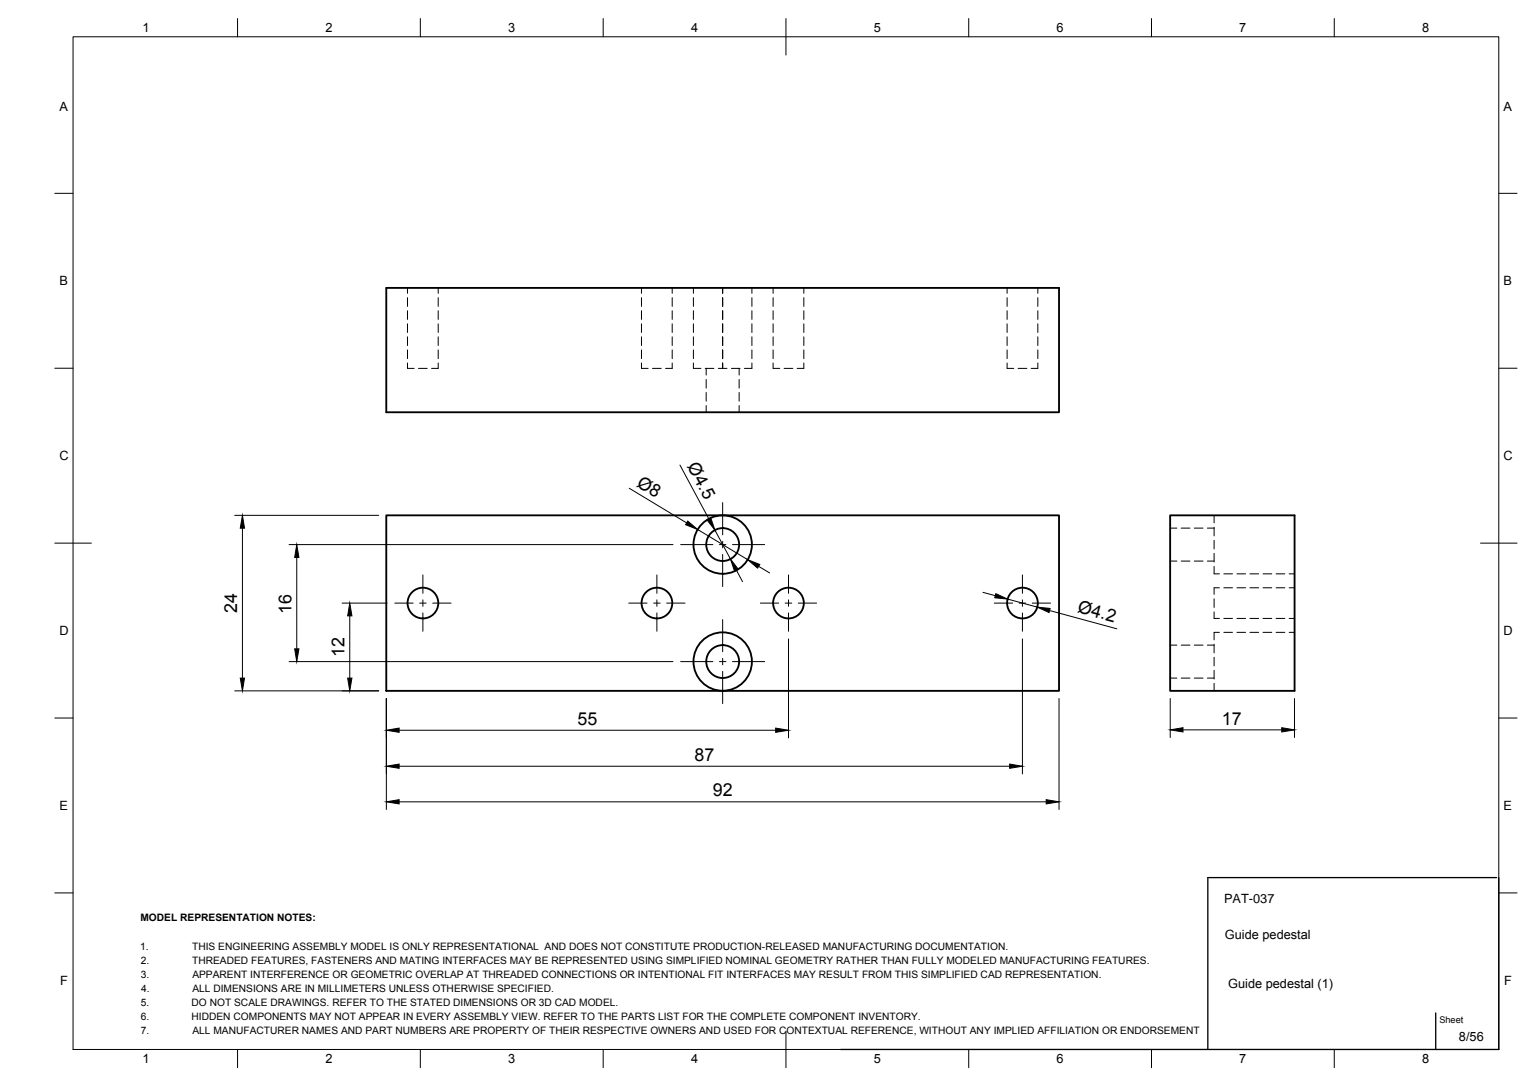
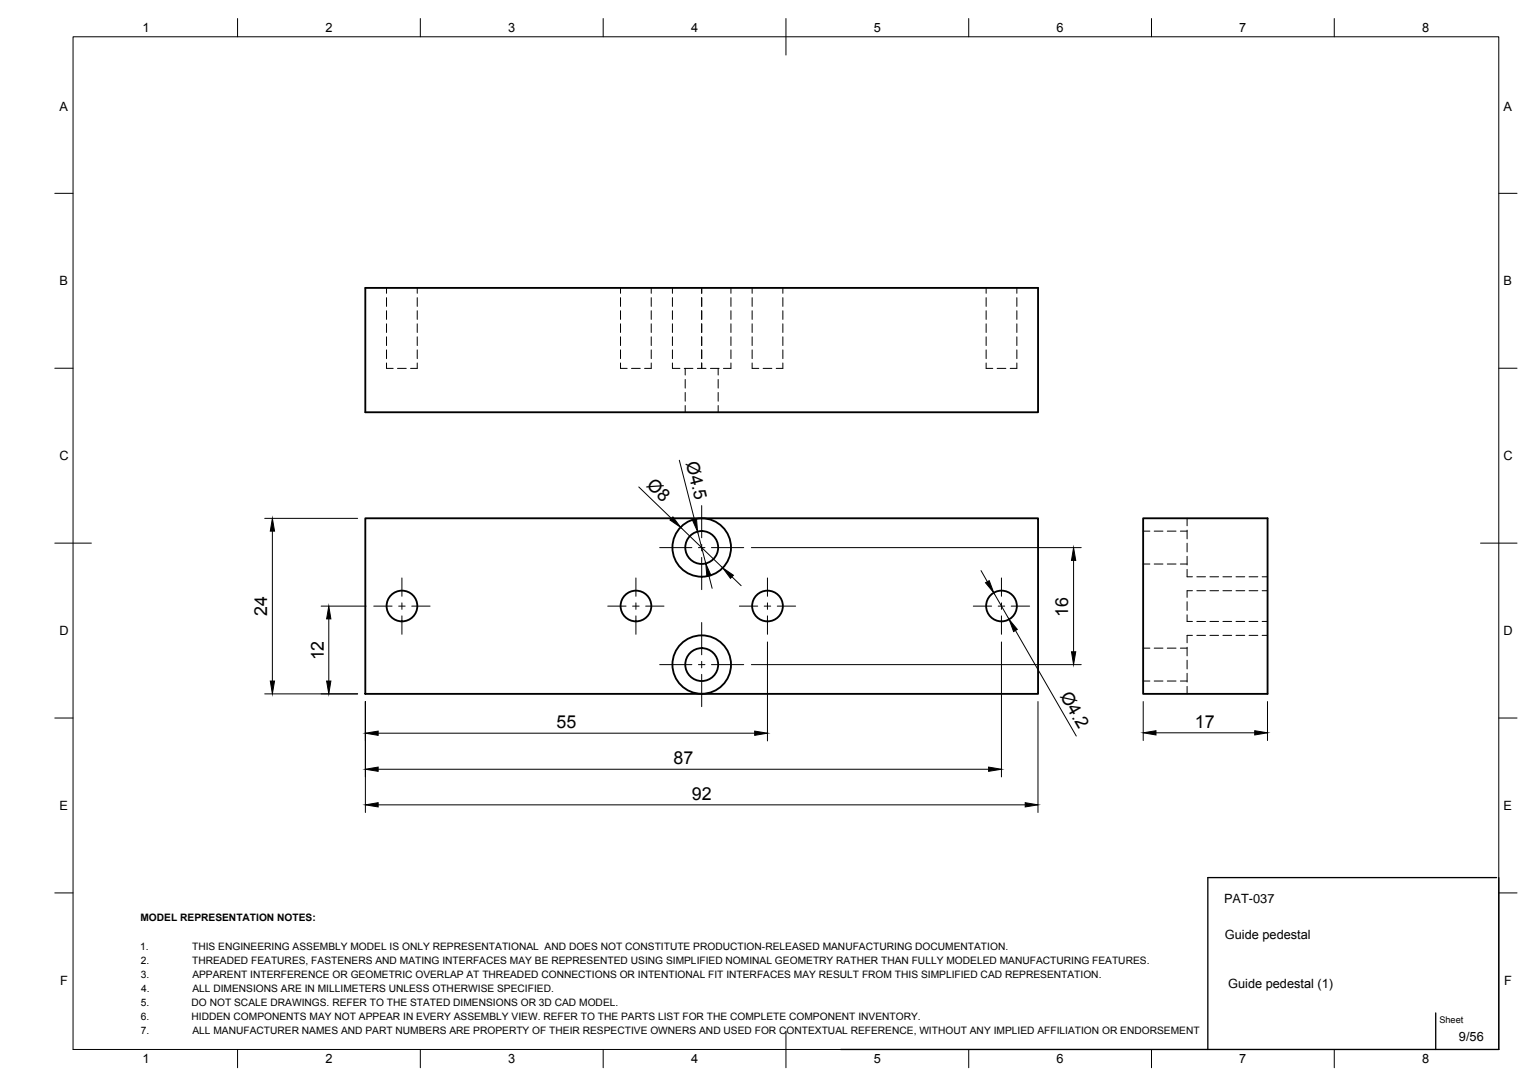
ISO-10303-21;
HEADER;
/* Generated by software containing ST-Developer
 * from STEP Tools, Inc. (www.steptools.com) 
 */

FILE_DESCRIPTION(
/* description */ ('Flywheel Crank-Slider'),
/* implementation_level */ '2;1');

FILE_NAME(
/* name */ 'Guide pedestal.step',
/* time_stamp */ '2026-10-28T03:23:13-07:00',
/* author */ (''),
/* organization */ (''),
/* preprocessor_version */ 'ST-DEVELOPER v20.2',
/* originating_system */ 'Autodesk Translation Framework v15.17.0.0',
/* authorisation */ '');

FILE_SCHEMA (('AUTOMOTIVE_DESIGN { 1 0 10303 214 3 1 1 }'));
ENDSEC;

DATA;
#10=MECHANICAL_DESIGN_GEOMETRIC_PRESENTATION_REPRESENTATION('',(#675),#17322);
#571=SHAPE_REPRESENTATION_RELATIONSHIP('SRR','None',#17567,#623);
#623=ADVANCED_BREP_SHAPE_REPRESENTATION('',(#736),#17271);
#675=STYLED_ITEM('',(#17945),#736);
#736=MANIFOLD_SOLID_BREP('Body1',#9053);
#845=FACE_BOUND('',#1996,.T.);
#846=FACE_BOUND('',#1999,.T.);
#847=FACE_BOUND('',#2001,.T.);
#848=FACE_BOUND('',#2002,.T.);
#849=FACE_BOUND('',#2003,.T.);
#850=FACE_BOUND('',#2004,.T.);
#851=FACE_BOUND('',#2020,.T.);
#852=FACE_BOUND('',#2021,.T.);
#1049=PLANE('',#9859);
#1050=PLANE('',#9864);
#1051=PLANE('',#9866);
#1052=PLANE('',#9877);
#1053=PLANE('',#9880);
#1054=PLANE('',#9883);
#1055=PLANE('',#9886);
#1056=PLANE('',#9887);
#1057=PLANE('',#9888);
#1058=PLANE('',#9889);
#1059=PLANE('',#9890);
#1060=PLANE('',#9891);
#1398=FACE_OUTER_BOUND('',#1993,.T.);
#1399=FACE_OUTER_BOUND('',#1994,.T.);
#1400=FACE_OUTER_BOUND('',#1995,.T.);
#1401=FACE_OUTER_BOUND('',#1997,.T.);
#1402=FACE_OUTER_BOUND('',#1998,.T.);
#1403=FACE_OUTER_BOUND('',#2000,.T.);
#1404=FACE_OUTER_BOUND('',#2005,.T.);
#1405=FACE_OUTER_BOUND('',#2006,.T.);
#1406=FACE_OUTER_BOUND('',#2007,.T.);
#1407=FACE_OUTER_BOUND('',#2008,.T.);
#1408=FACE_OUTER_BOUND('',#2009,.T.);
#1409=FACE_OUTER_BOUND('',#2010,.T.);
#1410=FACE_OUTER_BOUND('',#2011,.T.);
#1411=FACE_OUTER_BOUND('',#2012,.T.);
#1412=FACE_OUTER_BOUND('',#2013,.T.);
#1413=FACE_OUTER_BOUND('',#2014,.T.);
#1414=FACE_OUTER_BOUND('',#2015,.T.);
#1415=FACE_OUTER_BOUND('',#2016,.T.);
#1416=FACE_OUTER_BOUND('',#2017,.T.);
#1417=FACE_OUTER_BOUND('',#2018,.T.);
#1418=FACE_OUTER_BOUND('',#2019,.T.);
#1993=EDGE_LOOP('',(#6434,#6435,#6436,#6437));
#1994=EDGE_LOOP('',(#6438,#6439,#6440,#6441));
#1995=EDGE_LOOP('',(#6442));
#1996=EDGE_LOOP('',(#6443));
#1997=EDGE_LOOP('',(#6444,#6445,#6446,#6447));
#1998=EDGE_LOOP('',(#6448,#6449));
#1999=EDGE_LOOP('',(#6450));
#2000=EDGE_LOOP('',(#6451,#6452,#6453,#6454,#6455,#6456,#6457,#6458,#6459));
#2001=EDGE_LOOP('',(#6460));
#2002=EDGE_LOOP('',(#6461));
#2003=EDGE_LOOP('',(#6462));
#2004=EDGE_LOOP('',(#6463));
#2005=EDGE_LOOP('',(#6464,#6465,#6466,#6467));
#2006=EDGE_LOOP('',(#6468,#6469,#6470,#6471));
#2007=EDGE_LOOP('',(#6472,#6473,#6474,#6475));
#2008=EDGE_LOOP('',(#6476));
#2009=EDGE_LOOP('',(#6477,#6478,#6479,#6480));
#2010=EDGE_LOOP('',(#6481));
#2011=EDGE_LOOP('',(#6482,#6483,#6484,#6485));
#2012=EDGE_LOOP('',(#6486));
#2013=EDGE_LOOP('',(#6487,#6488,#6489,#6490));
#2014=EDGE_LOOP('',(#6491));
#2015=EDGE_LOOP('',(#6492,#6493,#6494,#6495));
#2016=EDGE_LOOP('',(#6496,#6497,#6498,#6499,#6500,#6501,#6502));
#2017=EDGE_LOOP('',(#6503,#6504,#6505,#6506));
#2018=EDGE_LOOP('',(#6507,#6508,#6509,#6510,#6511,#6512,#6513));
#2019=EDGE_LOOP('',(#6514,#6515,#6516,#6517));
#2020=EDGE_LOOP('',(#6518));
#2021=EDGE_LOOP('',(#6519));
#2692=LINE('',#14082,#3303);
#2693=LINE('',#14086,#3304);
#2694=LINE('',#14092,#3305);
#2695=LINE('',#14094,#3306);
#2696=LINE('',#14100,#3307);
#2697=LINE('',#14107,#3308);
#2698=LINE('',#14109,#3309);
#2699=LINE('',#14111,#3310);
#2700=LINE('',#14112,#3311);
#2701=LINE('',#14114,#3312);
#2702=LINE('',#14115,#3313);
#2703=LINE('',#14127,#3314);
#2704=LINE('',#14131,#3315);
#2705=LINE('',#14135,#3316);
#2706=LINE('',#14140,#3317);
#2707=LINE('',#14145,#3318);
#2708=LINE('',#14150,#3319);
#2709=LINE('',#14155,#3320);
#2710=LINE('',#14156,#3321);
#2711=LINE('',#14157,#3322);
#2712=LINE('',#14160,#3323);
#2713=LINE('',#14161,#3324);
#2714=LINE('',#14164,#3325);
#2715=LINE('',#14165,#3326);
#2716=LINE('',#14167,#3327);
#3303=VECTOR('',#11244,0.4);
#3304=VECTOR('',#11247,1.);
#3305=VECTOR('',#11254,1.);
#3306=VECTOR('',#11257,1.);
#3307=VECTOR('',#11266,1.);
#3308=VECTOR('',#11275,1.);
#3309=VECTOR('',#11276,1.);
#3310=VECTOR('',#11277,1.);
#3311=VECTOR('',#11278,1.);
#3312=VECTOR('',#11279,1.);
#3313=VECTOR('',#11280,1.);
#3314=VECTOR('',#11293,0.225);
#3315=VECTOR('',#11298,0.225);
#3316=VECTOR('',#11303,0.21);
#3317=VECTOR('',#11310,0.21);
#3318=VECTOR('',#11317,0.21);
#3319=VECTOR('',#11324,0.21);
#3320=VECTOR('',#11329,1.);
#3321=VECTOR('',#11330,1.);
#3322=VECTOR('',#11331,1.);
#3323=VECTOR('',#11334,1.);
#3324=VECTOR('',#11335,1.);
#3325=VECTOR('',#11338,1.);
#3326=VECTOR('',#11339,1.);
#3327=VECTOR('',#11342,1.);
#3918=CIRCLE('',#9854,0.4);
#3919=CIRCLE('',#9855,0.4);
#3920=CIRCLE('',#9857,0.4);
#3921=CIRCLE('',#9858,0.4);
#3922=CIRCLE('',#9860,0.225);
#3923=CIRCLE('',#9862,0.4);
#3924=CIRCLE('',#9863,0.4);
#3925=CIRCLE('',#9865,0.225);
#3926=CIRCLE('',#9867,0.21);
#3927=CIRCLE('',#9868,0.21);
#3928=CIRCLE('',#9869,0.21);
#3929=CIRCLE('',#9870,0.21);
#3930=CIRCLE('',#9872,0.225);
#3931=CIRCLE('',#9874,0.225);
#3932=CIRCLE('',#9876,0.21);
#3933=CIRCLE('',#9879,0.21);
#3934=CIRCLE('',#9882,0.21);
#3935=CIRCLE('',#9885,0.21);
#4381=VERTEX_POINT('',#14080);
#4382=VERTEX_POINT('',#14081);
#4383=VERTEX_POINT('',#14083);
#4384=VERTEX_POINT('',#14085);
#4385=VERTEX_POINT('',#14089);
#4386=VERTEX_POINT('',#14091);
#4387=VERTEX_POINT('',#14096);
#4388=VERTEX_POINT('',#14103);
#4389=VERTEX_POINT('',#14106);
#4390=VERTEX_POINT('',#14108);
#4391=VERTEX_POINT('',#14110);
#4392=VERTEX_POINT('',#14113);
#4393=VERTEX_POINT('',#14116);
#4394=VERTEX_POINT('',#14118);
#4395=VERTEX_POINT('',#14120);
#4396=VERTEX_POINT('',#14122);
#4397=VERTEX_POINT('',#14125);
#4398=VERTEX_POINT('',#14129);
#4399=VERTEX_POINT('',#14133);
#4400=VERTEX_POINT('',#14138);
#4401=VERTEX_POINT('',#14143);
#4402=VERTEX_POINT('',#14148);
#4403=VERTEX_POINT('',#14153);
#4404=VERTEX_POINT('',#14154);
#4405=VERTEX_POINT('',#14159);
#4406=VERTEX_POINT('',#14163);
#5174=EDGE_CURVE('',#4381,#4382,#2692,.T.);
#5175=EDGE_CURVE('',#4383,#4381,#3918,.T.);
#5176=EDGE_CURVE('',#4383,#4384,#2693,.T.);
#5177=EDGE_CURVE('',#4382,#4384,#3919,.T.);
#5178=EDGE_CURVE('',#4385,#4385,#3920,.T.);
#5179=EDGE_CURVE('',#4385,#4386,#2694,.T.);
#5180=EDGE_CURVE('',#4386,#4386,#3921,.T.);
#5181=EDGE_CURVE('',#4385,#4386,#2695,.T.);
#5182=EDGE_CURVE('',#4387,#4387,#3922,.T.);
#5183=EDGE_CURVE('',#4384,#4382,#3923,.T.);
#5184=EDGE_CURVE('',#4383,#4384,#2696,.T.);
#5185=EDGE_CURVE('',#4381,#4383,#3924,.T.);
#5186=EDGE_CURVE('',#4388,#4388,#3925,.T.);
#5187=EDGE_CURVE('',#4389,#4386,#2697,.T.);
#5188=EDGE_CURVE('',#4386,#4390,#2698,.T.);
#5189=EDGE_CURVE('',#4390,#4391,#2699,.T.);
#5190=EDGE_CURVE('',#4391,#4384,#2700,.T.);
#5191=EDGE_CURVE('',#4384,#4392,#2701,.T.);
#5192=EDGE_CURVE('',#4392,#4389,#2702,.T.);
#5193=EDGE_CURVE('',#4393,#4393,#3926,.T.);
#5194=EDGE_CURVE('',#4394,#4394,#3927,.T.);
#5195=EDGE_CURVE('',#4395,#4395,#3928,.T.);
#5196=EDGE_CURVE('',#4396,#4396,#3929,.T.);
#5197=EDGE_CURVE('',#4397,#4397,#3930,.T.);
#5198=EDGE_CURVE('',#4397,#4387,#2703,.T.);
#5199=EDGE_CURVE('',#4398,#4398,#3931,.T.);
#5200=EDGE_CURVE('',#4398,#4388,#2704,.T.);
#5201=EDGE_CURVE('',#4399,#4399,#3932,.T.);
#5202=EDGE_CURVE('',#4399,#4396,#2705,.T.);
#5203=EDGE_CURVE('',#4400,#4400,#3933,.T.);
#5204=EDGE_CURVE('',#4400,#4395,#2706,.T.);
#5205=EDGE_CURVE('',#4401,#4401,#3934,.T.);
#5206=EDGE_CURVE('',#4401,#4394,#2707,.T.);
#5207=EDGE_CURVE('',#4402,#4402,#3935,.T.);
#5208=EDGE_CURVE('',#4402,#4393,#2708,.T.);
#5209=EDGE_CURVE('',#4403,#4404,#2709,.T.);
#5210=EDGE_CURVE('',#4404,#4389,#2710,.T.);
#5211=EDGE_CURVE('',#4403,#4392,#2711,.T.);
#5212=EDGE_CURVE('',#4405,#4403,#2712,.T.);
#5213=EDGE_CURVE('',#4405,#4391,#2713,.T.);
#5214=EDGE_CURVE('',#4406,#4405,#2714,.T.);
#5215=EDGE_CURVE('',#4406,#4390,#2715,.T.);
#5216=EDGE_CURVE('',#4404,#4406,#2716,.T.);
#6434=ORIENTED_EDGE('',*,*,#5174,.F.);
#6435=ORIENTED_EDGE('',*,*,#5175,.F.);
#6436=ORIENTED_EDGE('',*,*,#5176,.T.);
#6437=ORIENTED_EDGE('',*,*,#5177,.F.);
#6438=ORIENTED_EDGE('',*,*,#5178,.F.);
#6439=ORIENTED_EDGE('',*,*,#5179,.T.);
#6440=ORIENTED_EDGE('',*,*,#5180,.F.);
#6441=ORIENTED_EDGE('',*,*,#5181,.F.);
#6442=ORIENTED_EDGE('',*,*,#5178,.T.);
#6443=ORIENTED_EDGE('',*,*,#5182,.F.);
#6444=ORIENTED_EDGE('',*,*,#5174,.T.);
#6445=ORIENTED_EDGE('',*,*,#5183,.F.);
#6446=ORIENTED_EDGE('',*,*,#5184,.F.);
#6447=ORIENTED_EDGE('',*,*,#5185,.F.);
#6448=ORIENTED_EDGE('',*,*,#5175,.T.);
#6449=ORIENTED_EDGE('',*,*,#5185,.T.);
#6450=ORIENTED_EDGE('',*,*,#5186,.F.);
#6451=ORIENTED_EDGE('',*,*,#5187,.T.);
#6452=ORIENTED_EDGE('',*,*,#5180,.T.);
#6453=ORIENTED_EDGE('',*,*,#5188,.T.);
#6454=ORIENTED_EDGE('',*,*,#5189,.T.);
#6455=ORIENTED_EDGE('',*,*,#5190,.T.);
#6456=ORIENTED_EDGE('',*,*,#5183,.T.);
#6457=ORIENTED_EDGE('',*,*,#5177,.T.);
#6458=ORIENTED_EDGE('',*,*,#5191,.T.);
#6459=ORIENTED_EDGE('',*,*,#5192,.T.);
#6460=ORIENTED_EDGE('',*,*,#5193,.T.);
#6461=ORIENTED_EDGE('',*,*,#5194,.T.);
#6462=ORIENTED_EDGE('',*,*,#5195,.T.);
#6463=ORIENTED_EDGE('',*,*,#5196,.T.);
#6464=ORIENTED_EDGE('',*,*,#5197,.F.);
#6465=ORIENTED_EDGE('',*,*,#5198,.T.);
#6466=ORIENTED_EDGE('',*,*,#5182,.T.);
#6467=ORIENTED_EDGE('',*,*,#5198,.F.);
#6468=ORIENTED_EDGE('',*,*,#5199,.F.);
#6469=ORIENTED_EDGE('',*,*,#5200,.T.);
#6470=ORIENTED_EDGE('',*,*,#5186,.T.);
#6471=ORIENTED_EDGE('',*,*,#5200,.F.);
#6472=ORIENTED_EDGE('',*,*,#5201,.F.);
#6473=ORIENTED_EDGE('',*,*,#5202,.T.);
#6474=ORIENTED_EDGE('',*,*,#5196,.F.);
#6475=ORIENTED_EDGE('',*,*,#5202,.F.);
#6476=ORIENTED_EDGE('',*,*,#5201,.T.);
#6477=ORIENTED_EDGE('',*,*,#5203,.F.);
#6478=ORIENTED_EDGE('',*,*,#5204,.T.);
#6479=ORIENTED_EDGE('',*,*,#5195,.F.);
#6480=ORIENTED_EDGE('',*,*,#5204,.F.);
#6481=ORIENTED_EDGE('',*,*,#5203,.T.);
#6482=ORIENTED_EDGE('',*,*,#5205,.F.);
#6483=ORIENTED_EDGE('',*,*,#5206,.T.);
#6484=ORIENTED_EDGE('',*,*,#5194,.F.);
#6485=ORIENTED_EDGE('',*,*,#5206,.F.);
#6486=ORIENTED_EDGE('',*,*,#5205,.T.);
#6487=ORIENTED_EDGE('',*,*,#5207,.F.);
#6488=ORIENTED_EDGE('',*,*,#5208,.T.);
#6489=ORIENTED_EDGE('',*,*,#5193,.F.);
#6490=ORIENTED_EDGE('',*,*,#5208,.F.);
#6491=ORIENTED_EDGE('',*,*,#5207,.T.);
#6492=ORIENTED_EDGE('',*,*,#5209,.T.);
#6493=ORIENTED_EDGE('',*,*,#5210,.T.);
#6494=ORIENTED_EDGE('',*,*,#5192,.F.);
#6495=ORIENTED_EDGE('',*,*,#5211,.F.);
#6496=ORIENTED_EDGE('',*,*,#5212,.T.);
#6497=ORIENTED_EDGE('',*,*,#5211,.T.);
#6498=ORIENTED_EDGE('',*,*,#5191,.F.);
#6499=ORIENTED_EDGE('',*,*,#5176,.F.);
#6500=ORIENTED_EDGE('',*,*,#5184,.T.);
#6501=ORIENTED_EDGE('',*,*,#5190,.F.);
#6502=ORIENTED_EDGE('',*,*,#5213,.F.);
#6503=ORIENTED_EDGE('',*,*,#5214,.T.);
#6504=ORIENTED_EDGE('',*,*,#5213,.T.);
#6505=ORIENTED_EDGE('',*,*,#5189,.F.);
#6506=ORIENTED_EDGE('',*,*,#5215,.F.);
#6507=ORIENTED_EDGE('',*,*,#5216,.T.);
#6508=ORIENTED_EDGE('',*,*,#5215,.T.);
#6509=ORIENTED_EDGE('',*,*,#5188,.F.);
#6510=ORIENTED_EDGE('',*,*,#5179,.F.);
#6511=ORIENTED_EDGE('',*,*,#5181,.T.);
#6512=ORIENTED_EDGE('',*,*,#5187,.F.);
#6513=ORIENTED_EDGE('',*,*,#5210,.F.);
#6514=ORIENTED_EDGE('',*,*,#5216,.F.);
#6515=ORIENTED_EDGE('',*,*,#5209,.F.);
#6516=ORIENTED_EDGE('',*,*,#5212,.F.);
#6517=ORIENTED_EDGE('',*,*,#5214,.F.);
#6518=ORIENTED_EDGE('',*,*,#5197,.T.);
#6519=ORIENTED_EDGE('',*,*,#5199,.T.);
#8370=CYLINDRICAL_SURFACE('',#9853,0.4);
#8371=CYLINDRICAL_SURFACE('',#9856,0.4);
#8372=CYLINDRICAL_SURFACE('',#9861,0.4);
#8373=CYLINDRICAL_SURFACE('',#9871,0.225);
#8374=CYLINDRICAL_SURFACE('',#9873,0.225);
#8375=CYLINDRICAL_SURFACE('',#9875,0.21);
#8376=CYLINDRICAL_SURFACE('',#9878,0.21);
#8377=CYLINDRICAL_SURFACE('',#9881,0.21);
#8378=CYLINDRICAL_SURFACE('',#9884,0.21);
#8589=ADVANCED_FACE('',(#1398),#8370,.F.);
#8590=ADVANCED_FACE('',(#1399),#8371,.F.);
#8591=ADVANCED_FACE('',(#1400,#845),#1049,.T.);
#8592=ADVANCED_FACE('',(#1401),#8372,.F.);
#8593=ADVANCED_FACE('',(#1402,#846),#1050,.T.);
#8594=ADVANCED_FACE('',(#1403,#847,#848,#849,#850),#1051,.T.);
#8595=ADVANCED_FACE('',(#1404),#8373,.F.);
#8596=ADVANCED_FACE('',(#1405),#8374,.F.);
#8597=ADVANCED_FACE('',(#1406),#8375,.F.);
#8598=ADVANCED_FACE('',(#1407),#1052,.T.);
#8599=ADVANCED_FACE('',(#1408),#8376,.F.);
#8600=ADVANCED_FACE('',(#1409),#1053,.T.);
#8601=ADVANCED_FACE('',(#1410),#8377,.F.);
#8602=ADVANCED_FACE('',(#1411),#1054,.T.);
#8603=ADVANCED_FACE('',(#1412),#8378,.F.);
#8604=ADVANCED_FACE('',(#1413),#1055,.T.);
#8605=ADVANCED_FACE('',(#1414),#1056,.T.);
#8606=ADVANCED_FACE('',(#1415),#1057,.T.);
#8607=ADVANCED_FACE('',(#1416),#1058,.T.);
#8608=ADVANCED_FACE('',(#1417),#1059,.T.);
#8609=ADVANCED_FACE('',(#1418,#851,#852),#1060,.F.);
#9053=CLOSED_SHELL('',(#8589,#8590,#8591,#8592,#8593,#8594,#8595,#8596,
#8597,#8598,#8599,#8600,#8601,#8602,#8603,#8604,#8605,#8606,#8607,#8608,
#8609));
#9852=AXIS2_PLACEMENT_3D('',#14078,#11240,#11241);
#9853=AXIS2_PLACEMENT_3D('',#14079,#11242,#11243);
#9854=AXIS2_PLACEMENT_3D('',#14084,#11245,#11246);
#9855=AXIS2_PLACEMENT_3D('',#14087,#11248,#11249);
#9856=AXIS2_PLACEMENT_3D('',#14088,#11250,#11251);
#9857=AXIS2_PLACEMENT_3D('',#14090,#11252,#11253);
#9858=AXIS2_PLACEMENT_3D('',#14093,#11255,#11256);
#9859=AXIS2_PLACEMENT_3D('',#14095,#11258,#11259);
#9860=AXIS2_PLACEMENT_3D('',#14097,#11260,#11261);
#9861=AXIS2_PLACEMENT_3D('',#14098,#11262,#11263);
#9862=AXIS2_PLACEMENT_3D('',#14099,#11264,#11265);
#9863=AXIS2_PLACEMENT_3D('',#14101,#11267,#11268);
#9864=AXIS2_PLACEMENT_3D('',#14102,#11269,#11270);
#9865=AXIS2_PLACEMENT_3D('',#14104,#11271,#11272);
#9866=AXIS2_PLACEMENT_3D('',#14105,#11273,#11274);
#9867=AXIS2_PLACEMENT_3D('',#14117,#11281,#11282);
#9868=AXIS2_PLACEMENT_3D('',#14119,#11283,#11284);
#9869=AXIS2_PLACEMENT_3D('',#14121,#11285,#11286);
#9870=AXIS2_PLACEMENT_3D('',#14123,#11287,#11288);
#9871=AXIS2_PLACEMENT_3D('',#14124,#11289,#11290);
#9872=AXIS2_PLACEMENT_3D('',#14126,#11291,#11292);
#9873=AXIS2_PLACEMENT_3D('',#14128,#11294,#11295);
#9874=AXIS2_PLACEMENT_3D('',#14130,#11296,#11297);
#9875=AXIS2_PLACEMENT_3D('',#14132,#11299,#11300);
#9876=AXIS2_PLACEMENT_3D('',#14134,#11301,#11302);
#9877=AXIS2_PLACEMENT_3D('',#14136,#11304,#11305);
#9878=AXIS2_PLACEMENT_3D('',#14137,#11306,#11307);
#9879=AXIS2_PLACEMENT_3D('',#14139,#11308,#11309);
#9880=AXIS2_PLACEMENT_3D('',#14141,#11311,#11312);
#9881=AXIS2_PLACEMENT_3D('',#14142,#11313,#11314);
#9882=AXIS2_PLACEMENT_3D('',#14144,#11315,#11316);
#9883=AXIS2_PLACEMENT_3D('',#14146,#11318,#11319);
#9884=AXIS2_PLACEMENT_3D('',#14147,#11320,#11321);
#9885=AXIS2_PLACEMENT_3D('',#14149,#11322,#11323);
#9886=AXIS2_PLACEMENT_3D('',#14151,#11325,#11326);
#9887=AXIS2_PLACEMENT_3D('',#14152,#11327,#11328);
#9888=AXIS2_PLACEMENT_3D('',#14158,#11332,#11333);
#9889=AXIS2_PLACEMENT_3D('',#14162,#11336,#11337);
#9890=AXIS2_PLACEMENT_3D('',#14166,#11340,#11341);
#9891=AXIS2_PLACEMENT_3D('',#14168,#11343,#11344);
#11240=DIRECTION('axis',(0.,0.,1.));
#11241=DIRECTION('refdir',(1.,0.,0.));
#11242=DIRECTION('center_axis',(0.,0.,1.));
#11243=DIRECTION('ref_axis',(1.,0.,0.));
#11244=DIRECTION('',(0.,0.,1.));
#11245=DIRECTION('center_axis',(0.,0.,1.));
#11246=DIRECTION('ref_axis',(1.,0.,0.));
#11247=DIRECTION('',(0.,0.,1.));
#11248=DIRECTION('center_axis',(0.,0.,-1.));
#11249=DIRECTION('ref_axis',(1.,0.,0.));
#11250=DIRECTION('center_axis',(0.,0.,1.));
#11251=DIRECTION('ref_axis',(1.,0.,0.));
#11252=DIRECTION('center_axis',(0.,0.,1.));
#11253=DIRECTION('ref_axis',(1.,0.,0.));
#11254=DIRECTION('',(0.,0.,1.));
#11255=DIRECTION('center_axis',(0.,0.,-1.));
#11256=DIRECTION('ref_axis',(1.,0.,0.));
#11257=DIRECTION('',(0.,0.,1.));
#11258=DIRECTION('center_axis',(0.,0.,1.));
#11259=DIRECTION('ref_axis',(1.,0.,0.));
#11260=DIRECTION('center_axis',(0.,0.,1.));
#11261=DIRECTION('ref_axis',(1.,0.,0.));
#11262=DIRECTION('center_axis',(0.,0.,1.));
#11263=DIRECTION('ref_axis',(1.,0.,0.));
#11264=DIRECTION('center_axis',(0.,0.,-1.));
#11265=DIRECTION('ref_axis',(1.,0.,0.));
#11266=DIRECTION('',(0.,0.,1.));
#11267=DIRECTION('center_axis',(0.,0.,1.));
#11268=DIRECTION('ref_axis',(1.,0.,0.));
#11269=DIRECTION('center_axis',(0.,0.,1.));
#11270=DIRECTION('ref_axis',(1.,0.,0.));
#11271=DIRECTION('center_axis',(0.,0.,1.));
#11272=DIRECTION('ref_axis',(1.,0.,0.));
#11273=DIRECTION('center_axis',(0.,0.,1.));
#11274=DIRECTION('ref_axis',(1.,0.,0.));
#11275=DIRECTION('',(0.,-1.,0.));
#11276=DIRECTION('',(0.,-1.,0.));
#11277=DIRECTION('',(1.,0.,0.));
#11278=DIRECTION('',(0.,1.,0.));
#11279=DIRECTION('',(0.,1.,0.));
#11280=DIRECTION('',(-1.,0.,0.));
#11281=DIRECTION('center_axis',(0.,0.,-1.));
#11282=DIRECTION('ref_axis',(1.,0.,0.));
#11283=DIRECTION('center_axis',(0.,0.,-1.));
#11284=DIRECTION('ref_axis',(1.,0.,0.));
#11285=DIRECTION('center_axis',(0.,0.,-1.));
#11286=DIRECTION('ref_axis',(1.,0.,0.));
#11287=DIRECTION('center_axis',(0.,0.,-1.));
#11288=DIRECTION('ref_axis',(1.,0.,0.));
#11289=DIRECTION('center_axis',(0.,0.,1.));
#11290=DIRECTION('ref_axis',(1.,0.,0.));
#11291=DIRECTION('center_axis',(0.,0.,1.));
#11292=DIRECTION('ref_axis',(1.,0.,0.));
#11293=DIRECTION('',(0.,0.,1.));
#11294=DIRECTION('center_axis',(0.,0.,1.));
#11295=DIRECTION('ref_axis',(1.,0.,0.));
#11296=DIRECTION('center_axis',(0.,0.,1.));
#11297=DIRECTION('ref_axis',(1.,0.,0.));
#11298=DIRECTION('',(0.,0.,1.));
#11299=DIRECTION('center_axis',(0.,0.,1.));
#11300=DIRECTION('ref_axis',(1.,0.,0.));
#11301=DIRECTION('center_axis',(0.,0.,1.));
#11302=DIRECTION('ref_axis',(1.,0.,0.));
#11303=DIRECTION('',(0.,0.,1.));
#11304=DIRECTION('center_axis',(0.,0.,1.));
#11305=DIRECTION('ref_axis',(1.,0.,0.));
#11306=DIRECTION('center_axis',(0.,0.,1.));
#11307=DIRECTION('ref_axis',(1.,0.,0.));
#11308=DIRECTION('center_axis',(0.,0.,1.));
#11309=DIRECTION('ref_axis',(1.,0.,0.));
#11310=DIRECTION('',(0.,0.,1.));
#11311=DIRECTION('center_axis',(0.,0.,1.));
#11312=DIRECTION('ref_axis',(1.,0.,0.));
#11313=DIRECTION('center_axis',(0.,0.,1.));
#11314=DIRECTION('ref_axis',(1.,0.,0.));
#11315=DIRECTION('center_axis',(0.,0.,1.));
#11316=DIRECTION('ref_axis',(1.,0.,0.));
#11317=DIRECTION('',(0.,0.,1.));
#11318=DIRECTION('center_axis',(0.,0.,1.));
#11319=DIRECTION('ref_axis',(1.,0.,0.));
#11320=DIRECTION('center_axis',(0.,0.,1.));
#11321=DIRECTION('ref_axis',(1.,0.,0.));
#11322=DIRECTION('center_axis',(0.,0.,1.));
#11323=DIRECTION('ref_axis',(1.,0.,0.));
#11324=DIRECTION('',(0.,0.,1.));
#11325=DIRECTION('center_axis',(0.,0.,1.));
#11326=DIRECTION('ref_axis',(1.,0.,0.));
#11327=DIRECTION('center_axis',(0.,1.,0.));
#11328=DIRECTION('ref_axis',(-1.,0.,0.));
#11329=DIRECTION('',(-1.,0.,0.));
#11330=DIRECTION('',(0.,0.,1.));
#11331=DIRECTION('',(0.,0.,1.));
#11332=DIRECTION('center_axis',(1.,0.,0.));
#11333=DIRECTION('ref_axis',(0.,1.,0.));
#11334=DIRECTION('',(0.,1.,0.));
#11335=DIRECTION('',(0.,0.,1.));
#11336=DIRECTION('center_axis',(0.,-1.,0.));
#11337=DIRECTION('ref_axis',(1.,0.,0.));
#11338=DIRECTION('',(1.,0.,0.));
#11339=DIRECTION('',(0.,0.,1.));
#11340=DIRECTION('center_axis',(-1.,0.,0.));
#11341=DIRECTION('ref_axis',(0.,-1.,0.));
#11342=DIRECTION('',(0.,-1.,0.));
#11343=DIRECTION('center_axis',(0.,0.,1.));
#11344=DIRECTION('ref_axis',(1.,0.,0.));
#14078=CARTESIAN_POINT('',(0.,0.,0.));
#14079=CARTESIAN_POINT('Origin',(4.8,0.,1.6));
#14080=CARTESIAN_POINT('',(4.4,-4.89858719658942E-17,1.6));
#14081=CARTESIAN_POINT('',(4.4,-4.89858719658942E-17,2.7));
#14082=CARTESIAN_POINT('',(4.4,-4.89858719658942E-17,1.6));
#14083=CARTESIAN_POINT('',(5.2,0.,1.6));
#14084=CARTESIAN_POINT('Origin',(4.8,0.,1.6));
#14085=CARTESIAN_POINT('',(5.2,0.,2.7));
#14086=CARTESIAN_POINT('',(5.2,0.,1.6));
#14087=CARTESIAN_POINT('Origin',(4.8,0.,2.7));
#14088=CARTESIAN_POINT('Origin',(3.2,0.,1.6));
#14089=CARTESIAN_POINT('',(2.8,-4.89858719658941E-17,1.6));
#14090=CARTESIAN_POINT('Origin',(3.2,0.,1.6));
#14091=CARTESIAN_POINT('',(2.8,0.,2.7));
#14092=CARTESIAN_POINT('',(2.8,0.,1.6));
#14093=CARTESIAN_POINT('Origin',(3.2,0.,2.7));
#14094=CARTESIAN_POINT('',(2.8,0.,1.6));
#14095=CARTESIAN_POINT('Origin',(3.2,0.,1.6));
#14096=CARTESIAN_POINT('',(2.975,-2.75545529808155E-17,1.6));
#14097=CARTESIAN_POINT('Origin',(3.2,0.,1.6));
#14098=CARTESIAN_POINT('Origin',(4.8,0.,1.6));
#14099=CARTESIAN_POINT('Origin',(4.8,0.,2.7));
#14100=CARTESIAN_POINT('',(5.2,0.,1.6));
#14101=CARTESIAN_POINT('Origin',(4.8,0.,1.6));
#14102=CARTESIAN_POINT('Origin',(4.8,0.,1.6));
#14103=CARTESIAN_POINT('',(4.575,-2.75545529808154E-17,1.6));
#14104=CARTESIAN_POINT('Origin',(4.8,0.,1.6));
#14105=CARTESIAN_POINT('Origin',(4.,0.,2.7));
#14106=CARTESIAN_POINT('',(2.8,4.6,2.7));
#14107=CARTESIAN_POINT('',(2.8,4.6,2.7));
#14108=CARTESIAN_POINT('',(2.8,-4.6,2.7));
#14109=CARTESIAN_POINT('',(2.8,4.6,2.7));
#14110=CARTESIAN_POINT('',(5.2,-4.6,2.7));
#14111=CARTESIAN_POINT('',(2.8,-4.6,2.7));
#14112=CARTESIAN_POINT('',(5.2,-4.6,2.7));
#14113=CARTESIAN_POINT('',(5.2,4.6,2.7));
#14114=CARTESIAN_POINT('',(5.2,-4.6,2.7));
#14115=CARTESIAN_POINT('',(5.2,4.6,2.7));
#14116=CARTESIAN_POINT('',(3.79,4.1,2.7));
#14117=CARTESIAN_POINT('Origin',(4.,4.1,2.7));
#14118=CARTESIAN_POINT('',(3.79,-4.1,2.7));
#14119=CARTESIAN_POINT('Origin',(4.,-4.1,2.7));
#14120=CARTESIAN_POINT('',(3.79,-0.9,2.7));
#14121=CARTESIAN_POINT('Origin',(4.,-0.9,2.7));
#14122=CARTESIAN_POINT('',(3.79,0.9,2.7));
#14123=CARTESIAN_POINT('Origin',(4.,0.9,2.7));
#14124=CARTESIAN_POINT('Origin',(3.2,0.,0.9));
#14125=CARTESIAN_POINT('',(2.975,-2.75545529808155E-17,1.));
#14126=CARTESIAN_POINT('Origin',(3.2,0.,1.));
#14127=CARTESIAN_POINT('',(2.975,-2.75545529808155E-17,0.9));
#14128=CARTESIAN_POINT('Origin',(4.8,0.,0.9));
#14129=CARTESIAN_POINT('',(4.575,-2.75545529808154E-17,1.));
#14130=CARTESIAN_POINT('Origin',(4.8,0.,1.));
#14131=CARTESIAN_POINT('',(4.575,-2.75545529808154E-17,0.9));
#14132=CARTESIAN_POINT('Origin',(4.,0.9,1.6));
#14133=CARTESIAN_POINT('',(3.79,0.9,1.6));
#14134=CARTESIAN_POINT('Origin',(4.,0.9,1.6));
#14135=CARTESIAN_POINT('',(3.79,0.9,1.6));
#14136=CARTESIAN_POINT('Origin',(4.,0.9,1.6));
#14137=CARTESIAN_POINT('Origin',(4.,-0.9,1.6));
#14138=CARTESIAN_POINT('',(3.79,-0.9,1.6));
#14139=CARTESIAN_POINT('Origin',(4.,-0.9,1.6));
#14140=CARTESIAN_POINT('',(3.79,-0.9,1.6));
#14141=CARTESIAN_POINT('Origin',(4.,-0.9,1.6));
#14142=CARTESIAN_POINT('Origin',(4.,-4.1,1.6));
#14143=CARTESIAN_POINT('',(3.79,-4.1,1.6));
#14144=CARTESIAN_POINT('Origin',(4.,-4.1,1.6));
#14145=CARTESIAN_POINT('',(3.79,-4.1,1.6));
#14146=CARTESIAN_POINT('Origin',(4.,-4.1,1.6));
#14147=CARTESIAN_POINT('Origin',(4.,4.1,1.6));
#14148=CARTESIAN_POINT('',(3.79,4.1,1.6));
#14149=CARTESIAN_POINT('Origin',(4.,4.1,1.6));
#14150=CARTESIAN_POINT('',(3.79,4.1,1.6));
#14151=CARTESIAN_POINT('Origin',(4.,4.1,1.6));
#14152=CARTESIAN_POINT('Origin',(5.2,4.6,1.));
#14153=CARTESIAN_POINT('',(5.2,4.6,1.));
#14154=CARTESIAN_POINT('',(2.8,4.6,1.));
#14155=CARTESIAN_POINT('',(5.2,4.6,1.));
#14156=CARTESIAN_POINT('',(2.8,4.6,1.));
#14157=CARTESIAN_POINT('',(5.2,4.6,1.));
#14158=CARTESIAN_POINT('Origin',(5.2,-4.6,1.));
#14159=CARTESIAN_POINT('',(5.2,-4.6,1.));
#14160=CARTESIAN_POINT('',(5.2,-4.6,1.));
#14161=CARTESIAN_POINT('',(5.2,-4.6,1.));
#14162=CARTESIAN_POINT('Origin',(2.8,-4.6,1.));
#14163=CARTESIAN_POINT('',(2.8,-4.6,1.));
#14164=CARTESIAN_POINT('',(2.8,-4.6,1.));
#14165=CARTESIAN_POINT('',(2.8,-4.6,1.));
#14166=CARTESIAN_POINT('Origin',(2.8,4.6,1.));
#14167=CARTESIAN_POINT('',(2.8,4.6,1.));
#14168=CARTESIAN_POINT('Origin',(4.,0.,1.));
#17210=UNCERTAINTY_MEASURE_WITH_UNIT(LENGTH_MEASURE(0.001),#17323,
'DISTANCE_ACCURACY_VALUE',
'Maximum model space distance between geometric entities at asserted c
onnectivities');
#17261=UNCERTAINTY_MEASURE_WITH_UNIT(LENGTH_MEASURE(0.001),#17323,
'DISTANCE_ACCURACY_VALUE',
'Maximum model space distance between geometric entities at asserted c
onnectivities');
#17271=(
GEOMETRIC_REPRESENTATION_CONTEXT(3)
GLOBAL_UNCERTAINTY_ASSIGNED_CONTEXT((#17210))
GLOBAL_UNIT_ASSIGNED_CONTEXT((#17323,#17325,#17326))
REPRESENTATION_CONTEXT('','3D')
);
#17322=(
GEOMETRIC_REPRESENTATION_CONTEXT(3)
GLOBAL_UNCERTAINTY_ASSIGNED_CONTEXT((#17261))
GLOBAL_UNIT_ASSIGNED_CONTEXT((#17323,#17325,#17326))
REPRESENTATION_CONTEXT('','3D')
);
#17323=(
LENGTH_UNIT()
NAMED_UNIT(*)
SI_UNIT(.CENTI.,.METRE.)
);
#17325=(
NAMED_UNIT(*)
PLANE_ANGLE_UNIT()
SI_UNIT($,.RADIAN.)
);
#17326=(
NAMED_UNIT(*)
SI_UNIT($,.STERADIAN.)
SOLID_ANGLE_UNIT()
);
#17336=SHAPE_DEFINITION_REPRESENTATION(#17396,#17567);
#17396=PRODUCT_DEFINITION_SHAPE('',$,#17628);
#17567=SHAPE_REPRESENTATION('',(#9852),#17271);
#17618=PRODUCT_DEFINITION_CONTEXT('part definition',#17800,'design');
#17628=PRODUCT_DEFINITION('Guide pedestal','Guide pedestal',#17688,#17618);
#17688=PRODUCT_DEFINITION_FORMATION('',$,#17811);
#17800=APPLICATION_CONTEXT(
'Core Data for Automotive Mechanical Design Process');
#17801=PRODUCT_CONTEXT('part definition',#17800,'mechanical');
#17811=PRODUCT('Guide pedestal','Guide pedestal','Guide pedestal',(#17801));
#17939=COLOUR_RGB('Off White',0.89,0.88,0.83);
#17940=FILL_AREA_STYLE_COLOUR('',#17939);
#17941=FILL_AREA_STYLE('',(#17940));
#17942=SURFACE_STYLE_FILL_AREA(#17941);
#17943=SURFACE_SIDE_STYLE('',(#17942));
#17944=SURFACE_STYLE_USAGE(.BOTH.,#17943);
#17945=PRESENTATION_STYLE_ASSIGNMENT((#17944));
ENDSEC;
END-ISO-10303-21;
